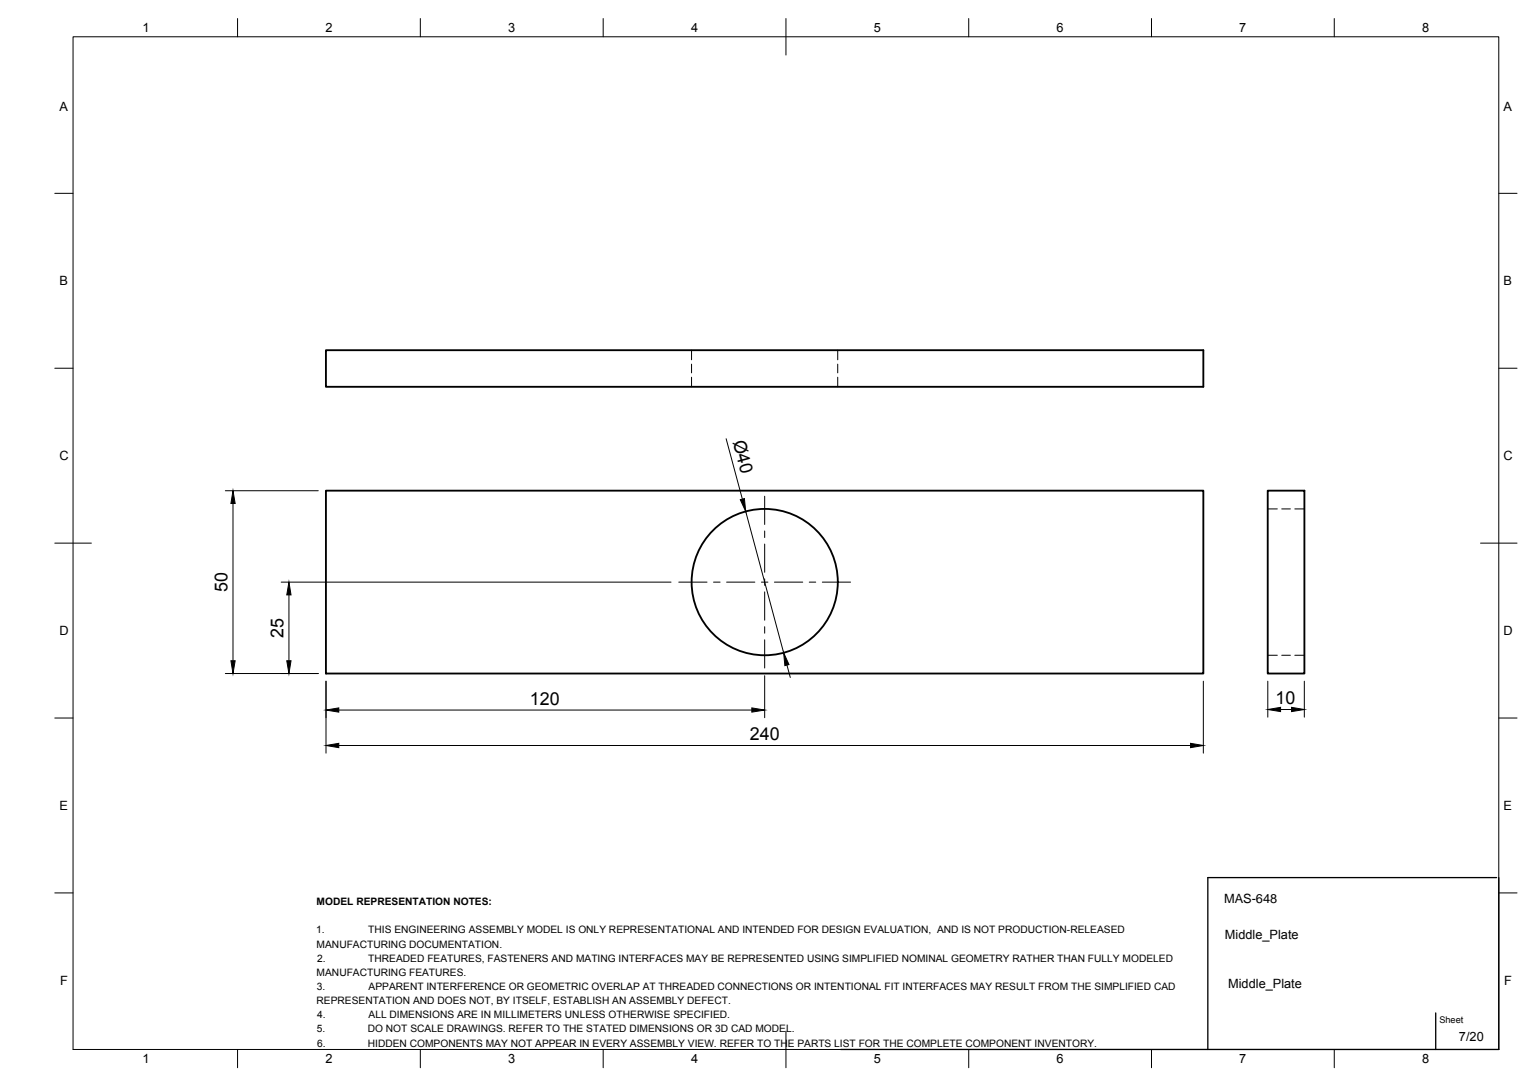
ISO-10303-21;
HEADER;
FILE_DESCRIPTION((''),'2;1');
FILE_NAME('Middle_Plate.step','2026-10-09T12:47:58-07:00',(''),(''),'','','');
FILE_SCHEMA (('AUTOMOTIVE_DESIGN { 1 0 10303 214 3 1 1 }'));
ENDSEC;
DATA;
#10=MECHANICAL_DESIGN_GEOMETRIC_PRESENTATION_REPRESENTATION('',(#311),#3475);
#141=FACE_BOUND('',#460,.T.) ;
#142=FACE_BOUND('',#462,.T.) ;
#166=CIRCLE('',#1980,20.) ;
#167=CIRCLE('',#1981,20.) ;
#256=CYLINDRICAL_SURFACE('',#1979,20.) ;
#287=SHAPE_REPRESENTATION_RELATIONSHIP('SRR','None',#3541,#299) ;
#299=ADVANCED_BREP_SHAPE_REPRESENTATION('',(#323),#3461) ;
#311=STYLED_ITEM('',(#3628),#323) ;
#323=MANIFOLD_SOLID_BREP('Body1',#1825) ;
#340=FACE_OUTER_BOUND('',#454,.T.) ;
#341=FACE_OUTER_BOUND('',#455,.T.) ;
#342=FACE_OUTER_BOUND('',#456,.T.) ;
#343=FACE_OUTER_BOUND('',#457,.T.) ;
#344=FACE_OUTER_BOUND('',#458,.T.) ;
#345=FACE_OUTER_BOUND('',#459,.T.) ;
#346=FACE_OUTER_BOUND('',#461,.T.) ;
#454=EDGE_LOOP('',(#1218,#1219,#1220,#1221)) ;
#455=EDGE_LOOP('',(#1222,#1223,#1224,#1225)) ;
#456=EDGE_LOOP('',(#1226,#1227,#1228,#1229)) ;
#457=EDGE_LOOP('',(#1230,#1231,#1232,#1233)) ;
#458=EDGE_LOOP('',(#1234,#1235,#1236,#1237)) ;
#459=EDGE_LOOP('',(#1238,#1239,#1240,#1241)) ;
#460=EDGE_LOOP('',(#1242)) ;
#461=EDGE_LOOP('',(#1243,#1244,#1245,#1246)) ;
#462=EDGE_LOOP('',(#1247)) ;
#599=LINE('',#2857,#718) ;
#600=LINE('',#2862,#719) ;
#601=LINE('',#2864,#720) ;
#602=LINE('',#2866,#721) ;
#603=LINE('',#2867,#722) ;
#604=LINE('',#2870,#723) ;
#605=LINE('',#2872,#724) ;
#606=LINE('',#2873,#725) ;
#607=LINE('',#2876,#726) ;
#608=LINE('',#2878,#727) ;
#609=LINE('',#2879,#728) ;
#610=LINE('',#2881,#729) ;
#611=LINE('',#2882,#730) ;
#718=VECTOR('',#2250,20.) ;
#719=VECTOR('',#2255,1000.) ;
#720=VECTOR('',#2256,1000.) ;
#721=VECTOR('',#2257,1000.) ;
#722=VECTOR('',#2258,1000.) ;
#723=VECTOR('',#2261,1000.) ;
#724=VECTOR('',#2262,1000.) ;
#725=VECTOR('',#2263,1000.) ;
#726=VECTOR('',#2266,1000.) ;
#727=VECTOR('',#2267,1000.) ;
#728=VECTOR('',#2268,1000.) ;
#729=VECTOR('',#2271,1000.) ;
#730=VECTOR('',#2272,1000.) ;
#833=VERTEX_POINT('',#2854) ;
#834=VERTEX_POINT('',#2856) ;
#835=VERTEX_POINT('',#2860) ;
#836=VERTEX_POINT('',#2861) ;
#837=VERTEX_POINT('',#2863) ;
#838=VERTEX_POINT('',#2865) ;
#839=VERTEX_POINT('',#2869) ;
#840=VERTEX_POINT('',#2871) ;
#841=VERTEX_POINT('',#2875) ;
#842=VERTEX_POINT('',#2877) ;
#981=EDGE_CURVE('',#833,#833,#166,.T.) ;
#982=EDGE_CURVE('',#833,#834,#599,.T.) ;
#983=EDGE_CURVE('',#834,#834,#167,.T.) ;
#984=EDGE_CURVE('',#835,#836,#600,.T.) ;
#985=EDGE_CURVE('',#837,#835,#601,.T.) ;
#986=EDGE_CURVE('',#837,#838,#602,.T.) ;
#987=EDGE_CURVE('',#838,#836,#603,.T.) ;
#988=EDGE_CURVE('',#839,#835,#604,.T.) ;
#989=EDGE_CURVE('',#840,#839,#605,.T.) ;
#990=EDGE_CURVE('',#840,#837,#606,.T.) ;
#991=EDGE_CURVE('',#841,#839,#607,.T.) ;
#992=EDGE_CURVE('',#842,#841,#608,.T.) ;
#993=EDGE_CURVE('',#842,#840,#609,.T.) ;
#994=EDGE_CURVE('',#836,#841,#610,.T.) ;
#995=EDGE_CURVE('',#838,#842,#611,.T.) ;
#1218=ORIENTED_EDGE('',*,*,#981,.F.) ;
#1219=ORIENTED_EDGE('',*,*,#982,.T.) ;
#1220=ORIENTED_EDGE('',*,*,#983,.T.) ;
#1221=ORIENTED_EDGE('',*,*,#982,.F.) ;
#1222=ORIENTED_EDGE('',*,*,#984,.F.) ;
#1223=ORIENTED_EDGE('',*,*,#985,.F.) ;
#1224=ORIENTED_EDGE('',*,*,#986,.T.) ;
#1225=ORIENTED_EDGE('',*,*,#987,.T.) ;
#1226=ORIENTED_EDGE('',*,*,#988,.F.) ;
#1227=ORIENTED_EDGE('',*,*,#989,.F.) ;
#1228=ORIENTED_EDGE('',*,*,#990,.T.) ;
#1229=ORIENTED_EDGE('',*,*,#985,.T.) ;
#1230=ORIENTED_EDGE('',*,*,#991,.F.) ;
#1231=ORIENTED_EDGE('',*,*,#992,.F.) ;
#1232=ORIENTED_EDGE('',*,*,#993,.T.) ;
#1233=ORIENTED_EDGE('',*,*,#989,.T.) ;
#1234=ORIENTED_EDGE('',*,*,#994,.F.) ;
#1235=ORIENTED_EDGE('',*,*,#987,.F.) ;
#1236=ORIENTED_EDGE('',*,*,#995,.T.) ;
#1237=ORIENTED_EDGE('',*,*,#992,.T.) ;
#1238=ORIENTED_EDGE('',*,*,#986,.F.) ;
#1239=ORIENTED_EDGE('',*,*,#990,.F.) ;
#1240=ORIENTED_EDGE('',*,*,#993,.F.) ;
#1241=ORIENTED_EDGE('',*,*,#995,.F.) ;
#1242=ORIENTED_EDGE('',*,*,#983,.F.) ;
#1243=ORIENTED_EDGE('',*,*,#984,.T.) ;
#1244=ORIENTED_EDGE('',*,*,#994,.T.) ;
#1245=ORIENTED_EDGE('',*,*,#991,.T.) ;
#1246=ORIENTED_EDGE('',*,*,#988,.T.) ;
#1247=ORIENTED_EDGE('',*,*,#981,.T.) ;
#1650=PLANE('',#1982) ;
#1651=PLANE('',#1983) ;
#1652=PLANE('',#1984) ;
#1653=PLANE('',#1985) ;
#1654=PLANE('',#1986) ;
#1655=PLANE('',#1987) ;
#1716=ADVANCED_FACE('',(#340),#256,.F.) ;
#1717=ADVANCED_FACE('',(#341),#1650,.T.) ;
#1718=ADVANCED_FACE('',(#342),#1651,.T.) ;
#1719=ADVANCED_FACE('',(#343),#1652,.T.) ;
#1720=ADVANCED_FACE('',(#344),#1653,.T.) ;
#1721=ADVANCED_FACE('',(#345,#141),#1654,.F.) ;
#1722=ADVANCED_FACE('',(#346,#142),#1655,.T.) ;
#1825=CLOSED_SHELL('',(#1716,#1717,#1718,#1719,#1720,#1721,#1722)) ;
#1978=AXIS2_PLACEMENT_3D('',#2852,#2244,#2245) ;
#1979=AXIS2_PLACEMENT_3D('',#2853,#2246,#2247) ;
#1980=AXIS2_PLACEMENT_3D('',#2855,#2248,#2249) ;
#1981=AXIS2_PLACEMENT_3D('',#2858,#2251,#2252) ;
#1982=AXIS2_PLACEMENT_3D('',#2859,#2253,#2254) ;
#1983=AXIS2_PLACEMENT_3D('',#2868,#2259,#2260) ;
#1984=AXIS2_PLACEMENT_3D('',#2874,#2264,#2265) ;
#1985=AXIS2_PLACEMENT_3D('',#2880,#2269,#2270) ;
#1986=AXIS2_PLACEMENT_3D('',#2883,#2273,#2274) ;
#1987=AXIS2_PLACEMENT_3D('',#2884,#2275,#2276) ;
#2244=DIRECTION('axis',(0.,0.,1.)) ;
#2245=DIRECTION('refdir',(1.,0.,0.)) ;
#2246=DIRECTION('center_axis',(0.,0.,-1.)) ;
#2247=DIRECTION('ref_axis',(-1.,0.,0.)) ;
#2248=DIRECTION('center_axis',(0.,0.,-1.)) ;
#2249=DIRECTION('ref_axis',(-1.,0.,0.)) ;
#2250=DIRECTION('',(0.,0.,-1.)) ;
#2251=DIRECTION('center_axis',(0.,0.,-1.)) ;
#2252=DIRECTION('ref_axis',(-1.,0.,0.)) ;
#2253=DIRECTION('center_axis',(-1.,0.,0.)) ;
#2254=DIRECTION('ref_axis',(0.,0.,1.)) ;
#2255=DIRECTION('',(0.,-1.,0.)) ;
#2256=DIRECTION('',(0.,0.,1.)) ;
#2257=DIRECTION('',(0.,-1.,0.)) ;
#2258=DIRECTION('',(0.,0.,1.)) ;
#2259=DIRECTION('center_axis',(-1.30104260698261E-16,1.,0.)) ;
#2260=DIRECTION('ref_axis',(-1.,-1.30104260698261E-16,0.)) ;
#2261=DIRECTION('',(-1.,-1.30104260698261E-16,0.)) ;
#2262=DIRECTION('',(0.,0.,1.)) ;
#2263=DIRECTION('',(-1.,-1.30104260698261E-16,0.)) ;
#2264=DIRECTION('center_axis',(1.,0.,0.)) ;
#2265=DIRECTION('ref_axis',(0.,0.,-1.)) ;
#2266=DIRECTION('',(0.,1.,0.)) ;
#2267=DIRECTION('',(0.,0.,1.)) ;
#2268=DIRECTION('',(0.,1.,0.)) ;
#2269=DIRECTION('center_axis',(1.30104260698261E-16,-1.,0.)) ;
#2270=DIRECTION('ref_axis',(1.,1.30104260698261E-16,0.)) ;
#2271=DIRECTION('',(1.,1.30104260698261E-16,0.)) ;
#2272=DIRECTION('',(1.,1.30104260698261E-16,0.)) ;
#2273=DIRECTION('center_axis',(0.,0.,1.)) ;
#2274=DIRECTION('ref_axis',(1.,0.,0.)) ;
#2275=DIRECTION('center_axis',(0.,0.,1.)) ;
#2276=DIRECTION('ref_axis',(1.,0.,0.)) ;
#2852=CARTESIAN_POINT('',(0.,0.,0.)) ;
#2853=CARTESIAN_POINT('Origin',(-1.38777878078145E-14,3.46944695195361E-15,
0.)) ;
#2854=CARTESIAN_POINT('',(20.,1.02015335365891E-15,0.)) ;
#2855=CARTESIAN_POINT('Origin',(-1.38777878078145E-14,3.46944695195361E-15,
0.)) ;
#2856=CARTESIAN_POINT('',(20.,1.02015335365891E-15,-10.)) ;
#2857=CARTESIAN_POINT('',(20.,1.0201533536589E-15,0.)) ;
#2858=CARTESIAN_POINT('Origin',(-1.38777878078145E-14,3.46944695195361E-15,
-10.)) ;
#2859=CARTESIAN_POINT('Origin',(-120.,-25.,-10.)) ;
#2860=CARTESIAN_POINT('',(-120.,25.,0.)) ;
#2861=CARTESIAN_POINT('',(-120.,-25.,0.)) ;
#2862=CARTESIAN_POINT('',(-120.,-25.,0.)) ;
#2863=CARTESIAN_POINT('',(-120.,25.,-10.)) ;
#2864=CARTESIAN_POINT('',(-120.,25.,-10.)) ;
#2865=CARTESIAN_POINT('',(-120.,-25.,-10.)) ;
#2866=CARTESIAN_POINT('',(-120.,-25.,-10.)) ;
#2867=CARTESIAN_POINT('',(-120.,-25.,-10.)) ;
#2868=CARTESIAN_POINT('Origin',(120.,25.,-10.)) ;
#2869=CARTESIAN_POINT('',(120.,25.,0.)) ;
#2870=CARTESIAN_POINT('',(120.,25.,0.)) ;
#2871=CARTESIAN_POINT('',(120.,25.,-10.)) ;
#2872=CARTESIAN_POINT('',(120.,25.,-10.)) ;
#2873=CARTESIAN_POINT('',(120.,25.,-10.)) ;
#2874=CARTESIAN_POINT('Origin',(120.,-25.,-10.)) ;
#2875=CARTESIAN_POINT('',(120.,-25.,0.)) ;
#2876=CARTESIAN_POINT('',(120.,-25.,0.)) ;
#2877=CARTESIAN_POINT('',(120.,-25.,-10.)) ;
#2878=CARTESIAN_POINT('',(120.,-25.,-10.)) ;
#2879=CARTESIAN_POINT('',(120.,-25.,-10.)) ;
#2880=CARTESIAN_POINT('Origin',(120.,-25.,-10.)) ;
#2881=CARTESIAN_POINT('',(120.,-25.,0.)) ;
#2882=CARTESIAN_POINT('',(120.,-25.,-10.)) ;
#2883=CARTESIAN_POINT('Origin',(0.,0.,-10.)) ;
#2884=CARTESIAN_POINT('Origin',(0.,0.,0.)) ;
#3443=UNCERTAINTY_MEASURE_WITH_UNIT(LENGTH_MEASURE(0.01),#3476,
'DISTANCE_ACCURACY_VALUE',
'Maximum model space distance between geometric entities at asserted c
onnectivities') ;
#3457=UNCERTAINTY_MEASURE_WITH_UNIT(LENGTH_MEASURE(0.01),#3476,
'DISTANCE_ACCURACY_VALUE',
'Maximum model space distance between geometric entities at asserted c
onnectivities') ;
#3461=(
GEOMETRIC_REPRESENTATION_CONTEXT(3)
GLOBAL_UNCERTAINTY_ASSIGNED_CONTEXT((#3443))
GLOBAL_UNIT_ASSIGNED_CONTEXT((#3476,#3478,#3479))
REPRESENTATION_CONTEXT('','3D')
) ;
#3475=(
GEOMETRIC_REPRESENTATION_CONTEXT(3)
GLOBAL_UNCERTAINTY_ASSIGNED_CONTEXT((#3457))
GLOBAL_UNIT_ASSIGNED_CONTEXT((#3476,#3478,#3479))
REPRESENTATION_CONTEXT('','3D')
) ;
#3476=(
LENGTH_UNIT()
NAMED_UNIT(*)
SI_UNIT(.MILLI.,.METRE.)
) ;
#3478=(
NAMED_UNIT(*)
PLANE_ANGLE_UNIT()
SI_UNIT($,.RADIAN.)
) ;
#3479=(
NAMED_UNIT(*)
SI_UNIT($,.STERADIAN.)
SOLID_ANGLE_UNIT()
) ;
#3483=SHAPE_DEFINITION_REPRESENTATION(#3500,#3541) ;
#3500=PRODUCT_DEFINITION_SHAPE('',$,#3559) ;
#3541=SHAPE_REPRESENTATION('',(#1978),#3461) ;
#3555=PRODUCT_DEFINITION_CONTEXT('part definition',#3608,'design') ;
#3559=PRODUCT_DEFINITION('Middle_Plate',
'Middle_Plate',#3576,#3555) ;
#3576=PRODUCT_DEFINITION_FORMATION('',$,#3613) ;
#3608=APPLICATION_CONTEXT(
'Core Data for Automotive Mechanical Design Process') ;
#3609=PRODUCT_CONTEXT('part definition',#3608,'mechanical') ;
#3613=PRODUCT('Middle_Plate',
'Middle_Plate',$,(#3609)) ;
#3628=PRESENTATION_STYLE_ASSIGNMENT((#3630)) ;
#3630=SURFACE_STYLE_USAGE(.BOTH.,#3632) ;
#3632=SURFACE_SIDE_STYLE('',(#3634)) ;
#3634=SURFACE_STYLE_FILL_AREA(#3636) ;
#3636=FILL_AREA_STYLE('Opaque(202,209,238)',(#3638)) ;
#3638=FILL_AREA_STYLE_COLOUR('Opaque(202,209,238)',#3640) ;
#3640=COLOUR_RGB('Opaque(202,209,238)', 0.09019608, 0.27058824, 0.51372549) ;
ENDSEC;
END-ISO-10303-21;
